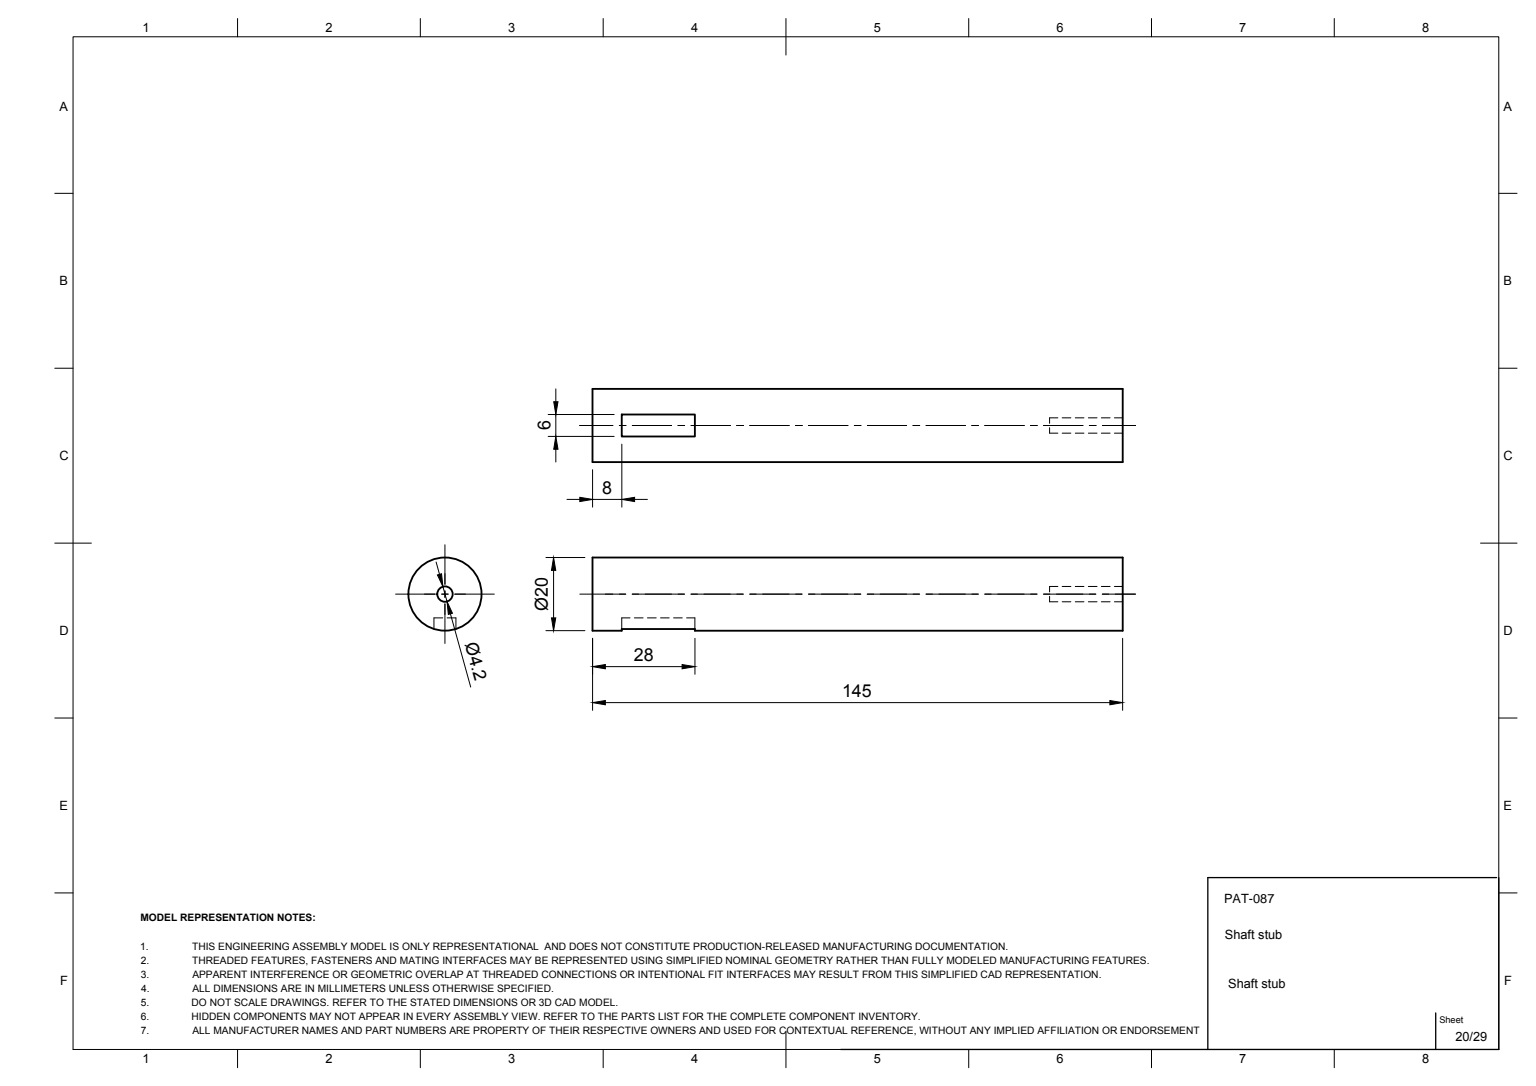
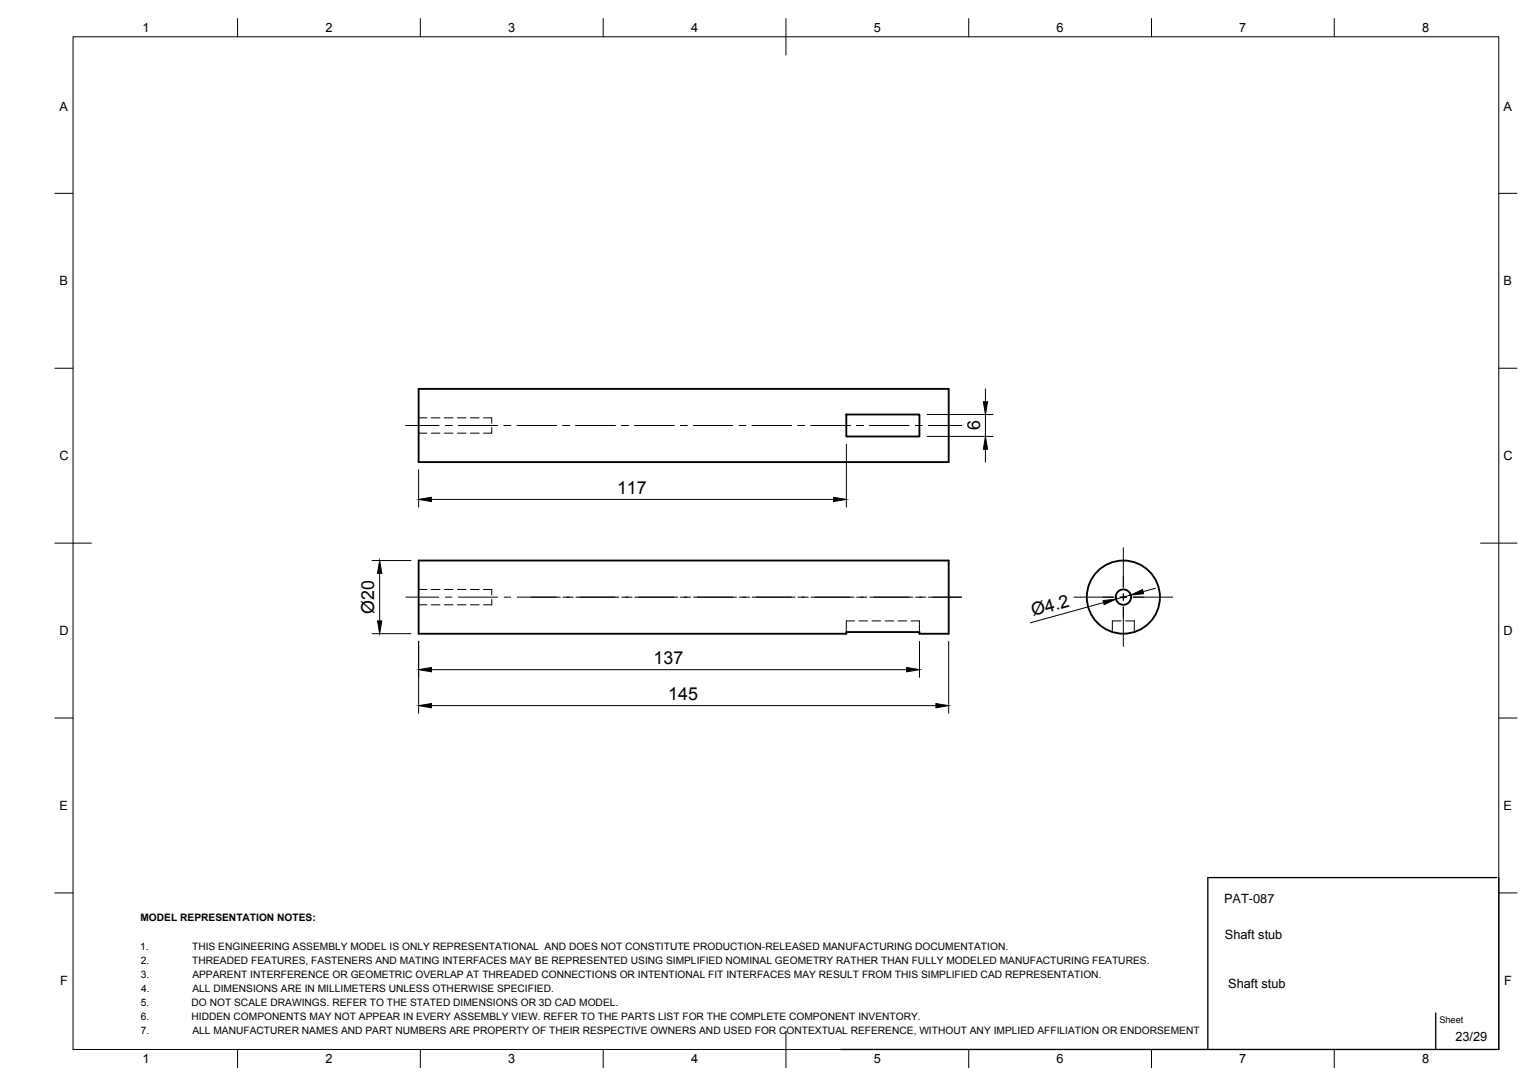
ISO-10303-21;
HEADER;
/* Generated by software containing ST-Developer
 * from STEP Tools, Inc. (www.steptools.com) 
 */

FILE_DESCRIPTION(
/* description */ ('Rigid flange shaft coupling assembly'),
/* implementation_level */ '2;1');

FILE_NAME(
/* name */ 'Shaft stub.step',
/* time_stamp */ '2026-10-27T10:47:16-07:00',
/* author */ (''),
/* organization */ (''),
/* preprocessor_version */ 'ST-DEVELOPER v20.2',
/* originating_system */ 'Autodesk Translation Framework v15.17.0.0',
/* authorisation */ '');

FILE_SCHEMA (('AUTOMOTIVE_DESIGN { 1 0 10303 214 3 1 1 }'));
ENDSEC;

DATA;
#10=MECHANICAL_DESIGN_GEOMETRIC_PRESENTATION_REPRESENTATION('',(#412),#9141);
#355=SHAPE_REPRESENTATION_RELATIONSHIP('SRR','None',#9291,#383);
#383=ADVANCED_BREP_SHAPE_REPRESENTATION('',(#440),#9126);
#412=STYLED_ITEM('',(#9500),#440);
#440=MANIFOLD_SOLID_BREP('Body1',#4767);
#517=FACE_BOUND('',#1207,.T.);
#518=FACE_BOUND('',#1210,.T.);
#645=PLANE('',#5312);
#646=PLANE('',#5313);
#647=PLANE('',#5314);
#648=PLANE('',#5316);
#649=PLANE('',#5317);
#650=PLANE('',#5318);
#651=PLANE('',#5323);
#652=PLANE('',#5324);
#863=FACE_OUTER_BOUND('',#1199,.T.);
#864=FACE_OUTER_BOUND('',#1200,.T.);
#865=FACE_OUTER_BOUND('',#1201,.T.);
#866=FACE_OUTER_BOUND('',#1202,.T.);
#867=FACE_OUTER_BOUND('',#1203,.T.);
#868=FACE_OUTER_BOUND('',#1204,.T.);
#869=FACE_OUTER_BOUND('',#1205,.T.);
#870=FACE_OUTER_BOUND('',#1206,.T.);
#871=FACE_OUTER_BOUND('',#1208,.T.);
#872=FACE_OUTER_BOUND('',#1209,.T.);
#1199=EDGE_LOOP('',(#3767,#3768,#3769,#3770));
#1200=EDGE_LOOP('',(#3771));
#1201=EDGE_LOOP('',(#3772,#3773,#3774,#3775));
#1202=EDGE_LOOP('',(#3776,#3777,#3778,#3779));
#1203=EDGE_LOOP('',(#3780,#3781,#3782,#3783));
#1204=EDGE_LOOP('',(#3784,#3785,#3786,#3787));
#1205=EDGE_LOOP('',(#3788,#3789,#3790,#3791));
#1206=EDGE_LOOP('',(#3792,#3793,#3794,#3795));
#1207=EDGE_LOOP('',(#3796,#3797,#3798,#3799));
#1208=EDGE_LOOP('',(#3800));
#1209=EDGE_LOOP('',(#3801));
#1210=EDGE_LOOP('',(#3802));
#1566=LINE('',#8079,#1911);
#1567=LINE('',#8085,#1912);
#1568=LINE('',#8087,#1913);
#1569=LINE('',#8089,#1914);
#1570=LINE('',#8090,#1915);
#1571=LINE('',#8095,#1916);
#1572=LINE('',#8096,#1917);
#1573=LINE('',#8099,#1918);
#1574=LINE('',#8101,#1919);
#1575=LINE('',#8102,#1920);
#1576=LINE('',#8104,#1921);
#1577=LINE('',#8111,#1922);
#1911=VECTOR('',#6239,0.21);
#1912=VECTOR('',#6246,1.);
#1913=VECTOR('',#6247,1.);
#1914=VECTOR('',#6248,1.);
#1915=VECTOR('',#6249,1.);
#1916=VECTOR('',#6254,1.);
#1917=VECTOR('',#6255,1.);
#1918=VECTOR('',#6258,1.);
#1919=VECTOR('',#6259,1.);
#1920=VECTOR('',#6260,1.);
#1921=VECTOR('',#6263,1.);
#1922=VECTOR('',#6272,1.);
#2172=CIRCLE('',#5310,0.21);
#2173=CIRCLE('',#5311,0.21);
#2174=CIRCLE('',#5315,1.);
#2175=CIRCLE('',#5319,1.);
#2176=CIRCLE('',#5321,1.);
#2177=CIRCLE('',#5322,1.);
#2457=VERTEX_POINT('',#8076);
#2458=VERTEX_POINT('',#8078);
#2459=VERTEX_POINT('',#8083);
#2460=VERTEX_POINT('',#8084);
#2461=VERTEX_POINT('',#8086);
#2462=VERTEX_POINT('',#8088);
#2463=VERTEX_POINT('',#8092);
#2464=VERTEX_POINT('',#8094);
#2465=VERTEX_POINT('',#8098);
#2466=VERTEX_POINT('',#8100);
#2467=VERTEX_POINT('',#8108);
#2468=VERTEX_POINT('',#8110);
#2927=EDGE_CURVE('',#2457,#2457,#2172,.T.);
#2928=EDGE_CURVE('',#2457,#2458,#1566,.T.);
#2929=EDGE_CURVE('',#2458,#2458,#2173,.T.);
#2930=EDGE_CURVE('',#2459,#2460,#1567,.T.);
#2931=EDGE_CURVE('',#2459,#2461,#1568,.T.);
#2932=EDGE_CURVE('',#2462,#2461,#1569,.T.);
#2933=EDGE_CURVE('',#2462,#2460,#1570,.T.);
#2934=EDGE_CURVE('',#2460,#2463,#2174,.T.);
#2935=EDGE_CURVE('',#2464,#2462,#1571,.T.);
#2936=EDGE_CURVE('',#2463,#2464,#1572,.T.);
#2937=EDGE_CURVE('',#2463,#2465,#1573,.T.);
#2938=EDGE_CURVE('',#2464,#2466,#1574,.T.);
#2939=EDGE_CURVE('',#2466,#2465,#1575,.T.);
#2940=EDGE_CURVE('',#2461,#2466,#1576,.T.);
#2941=EDGE_CURVE('',#2465,#2459,#2175,.T.);
#2942=EDGE_CURVE('',#2467,#2467,#2176,.T.);
#2943=EDGE_CURVE('',#2467,#2468,#1577,.T.);
#2944=EDGE_CURVE('',#2468,#2468,#2177,.T.);
#3767=ORIENTED_EDGE('',*,*,#2927,.F.);
#3768=ORIENTED_EDGE('',*,*,#2928,.T.);
#3769=ORIENTED_EDGE('',*,*,#2929,.T.);
#3770=ORIENTED_EDGE('',*,*,#2928,.F.);
#3771=ORIENTED_EDGE('',*,*,#2929,.F.);
#3772=ORIENTED_EDGE('',*,*,#2930,.F.);
#3773=ORIENTED_EDGE('',*,*,#2931,.T.);
#3774=ORIENTED_EDGE('',*,*,#2932,.F.);
#3775=ORIENTED_EDGE('',*,*,#2933,.T.);
#3776=ORIENTED_EDGE('',*,*,#2934,.F.);
#3777=ORIENTED_EDGE('',*,*,#2933,.F.);
#3778=ORIENTED_EDGE('',*,*,#2935,.F.);
#3779=ORIENTED_EDGE('',*,*,#2936,.F.);
#3780=ORIENTED_EDGE('',*,*,#2937,.F.);
#3781=ORIENTED_EDGE('',*,*,#2936,.T.);
#3782=ORIENTED_EDGE('',*,*,#2938,.T.);
#3783=ORIENTED_EDGE('',*,*,#2939,.T.);
#3784=ORIENTED_EDGE('',*,*,#2935,.T.);
#3785=ORIENTED_EDGE('',*,*,#2932,.T.);
#3786=ORIENTED_EDGE('',*,*,#2940,.T.);
#3787=ORIENTED_EDGE('',*,*,#2938,.F.);
#3788=ORIENTED_EDGE('',*,*,#2941,.F.);
#3789=ORIENTED_EDGE('',*,*,#2939,.F.);
#3790=ORIENTED_EDGE('',*,*,#2940,.F.);
#3791=ORIENTED_EDGE('',*,*,#2931,.F.);
#3792=ORIENTED_EDGE('',*,*,#2942,.F.);
#3793=ORIENTED_EDGE('',*,*,#2943,.T.);
#3794=ORIENTED_EDGE('',*,*,#2944,.T.);
#3795=ORIENTED_EDGE('',*,*,#2943,.F.);
#3796=ORIENTED_EDGE('',*,*,#2937,.T.);
#3797=ORIENTED_EDGE('',*,*,#2941,.T.);
#3798=ORIENTED_EDGE('',*,*,#2930,.T.);
#3799=ORIENTED_EDGE('',*,*,#2934,.T.);
#3800=ORIENTED_EDGE('',*,*,#2942,.T.);
#3801=ORIENTED_EDGE('',*,*,#2944,.F.);
#3802=ORIENTED_EDGE('',*,*,#2927,.T.);
#4438=CYLINDRICAL_SURFACE('',#5309,0.21);
#4439=CYLINDRICAL_SURFACE('',#5320,1.);
#4599=ADVANCED_FACE('',(#863),#4438,.F.);
#4600=ADVANCED_FACE('',(#864),#645,.F.);
#4601=ADVANCED_FACE('',(#865),#646,.F.);
#4602=ADVANCED_FACE('',(#866),#647,.T.);
#4603=ADVANCED_FACE('',(#867),#648,.F.);
#4604=ADVANCED_FACE('',(#868),#649,.F.);
#4605=ADVANCED_FACE('',(#869),#650,.F.);
#4606=ADVANCED_FACE('',(#870,#517),#4439,.T.);
#4607=ADVANCED_FACE('',(#871),#651,.T.);
#4608=ADVANCED_FACE('',(#872,#518),#652,.F.);
#4767=CLOSED_SHELL('',(#4599,#4600,#4601,#4602,#4603,#4604,#4605,#4606,
#4607,#4608));
#5308=AXIS2_PLACEMENT_3D('',#8074,#6233,#6234);
#5309=AXIS2_PLACEMENT_3D('',#8075,#6235,#6236);
#5310=AXIS2_PLACEMENT_3D('',#8077,#6237,#6238);
#5311=AXIS2_PLACEMENT_3D('',#8080,#6240,#6241);
#5312=AXIS2_PLACEMENT_3D('',#8081,#6242,#6243);
#5313=AXIS2_PLACEMENT_3D('',#8082,#6244,#6245);
#5314=AXIS2_PLACEMENT_3D('',#8091,#6250,#6251);
#5315=AXIS2_PLACEMENT_3D('',#8093,#6252,#6253);
#5316=AXIS2_PLACEMENT_3D('',#8097,#6256,#6257);
#5317=AXIS2_PLACEMENT_3D('',#8103,#6261,#6262);
#5318=AXIS2_PLACEMENT_3D('',#8105,#6264,#6265);
#5319=AXIS2_PLACEMENT_3D('',#8106,#6266,#6267);
#5320=AXIS2_PLACEMENT_3D('',#8107,#6268,#6269);
#5321=AXIS2_PLACEMENT_3D('',#8109,#6270,#6271);
#5322=AXIS2_PLACEMENT_3D('',#8112,#6273,#6274);
#5323=AXIS2_PLACEMENT_3D('',#8113,#6275,#6276);
#5324=AXIS2_PLACEMENT_3D('',#8114,#6277,#6278);
#6233=DIRECTION('axis',(0.,0.,1.));
#6234=DIRECTION('refdir',(1.,0.,0.));
#6235=DIRECTION('center_axis',(0.,1.,0.));
#6236=DIRECTION('ref_axis',(1.,0.,0.));
#6237=DIRECTION('center_axis',(0.,1.,0.));
#6238=DIRECTION('ref_axis',(1.,0.,0.));
#6239=DIRECTION('',(0.,1.,0.));
#6240=DIRECTION('center_axis',(0.,1.,0.));
#6241=DIRECTION('ref_axis',(1.,0.,0.));
#6242=DIRECTION('center_axis',(0.,1.,0.));
#6243=DIRECTION('ref_axis',(1.,0.,0.));
#6244=DIRECTION('center_axis',(-1.,0.,0.));
#6245=DIRECTION('ref_axis',(0.,0.,1.));
#6246=DIRECTION('',(0.,-1.,0.));
#6247=DIRECTION('',(0.,0.,1.));
#6248=DIRECTION('',(0.,1.,0.));
#6249=DIRECTION('',(0.,0.,-1.));
#6250=DIRECTION('center_axis',(0.,1.,0.));
#6251=DIRECTION('ref_axis',(1.,0.,0.));
#6252=DIRECTION('center_axis',(0.,-1.,0.));
#6253=DIRECTION('ref_axis',(1.,0.,0.));
#6254=DIRECTION('',(-1.,0.,0.));
#6255=DIRECTION('',(0.,0.,1.));
#6256=DIRECTION('center_axis',(1.,0.,0.));
#6257=DIRECTION('ref_axis',(0.,0.,-1.));
#6258=DIRECTION('',(0.,1.,0.));
#6259=DIRECTION('',(0.,1.,0.));
#6260=DIRECTION('',(0.,0.,-1.));
#6261=DIRECTION('center_axis',(0.,0.,1.));
#6262=DIRECTION('ref_axis',(1.,0.,0.));
#6263=DIRECTION('',(1.,0.,0.));
#6264=DIRECTION('center_axis',(0.,1.,0.));
#6265=DIRECTION('ref_axis',(0.,0.,1.));
#6266=DIRECTION('center_axis',(0.,1.,0.));
#6267=DIRECTION('ref_axis',(1.,0.,0.));
#6268=DIRECTION('center_axis',(0.,1.,0.));
#6269=DIRECTION('ref_axis',(1.,0.,0.));
#6270=DIRECTION('center_axis',(0.,1.,0.));
#6271=DIRECTION('ref_axis',(1.,0.,0.));
#6272=DIRECTION('',(0.,-1.,0.));
#6273=DIRECTION('center_axis',(0.,1.,0.));
#6274=DIRECTION('ref_axis',(1.,0.,0.));
#6275=DIRECTION('center_axis',(0.,1.,0.));
#6276=DIRECTION('ref_axis',(1.,0.,0.));
#6277=DIRECTION('center_axis',(0.,1.,0.));
#6278=DIRECTION('ref_axis',(1.,0.,0.));
#8074=CARTESIAN_POINT('',(0.,0.,0.));
#8075=CARTESIAN_POINT('Origin',(0.,-4.6,6.53));
#8076=CARTESIAN_POINT('',(-0.21,-4.5,6.53));
#8077=CARTESIAN_POINT('Origin',(0.,-4.5,6.53));
#8078=CARTESIAN_POINT('',(-0.21,-2.5,6.53));
#8079=CARTESIAN_POINT('',(-0.21,-4.6,6.53));
#8080=CARTESIAN_POINT('Origin',(0.,-2.5,6.53));
#8081=CARTESIAN_POINT('Origin',(0.,-2.5,6.53));
#8082=CARTESIAN_POINT('Origin',(-0.3,7.2,5.43));
#8083=CARTESIAN_POINT('',(-0.3,9.2,5.57606079858305));
#8084=CARTESIAN_POINT('',(-0.3,7.2,5.57606079858305));
#8085=CARTESIAN_POINT('',(-0.3,-4.5,5.57606079858305));
#8086=CARTESIAN_POINT('',(-0.3,9.2,5.88));
#8087=CARTESIAN_POINT('',(-0.3,9.2,5.88));
#8088=CARTESIAN_POINT('',(-0.3,7.2,5.88));
#8089=CARTESIAN_POINT('',(-0.3,7.2,5.88));
#8090=CARTESIAN_POINT('',(-0.3,7.2,5.88));
#8091=CARTESIAN_POINT('Origin',(0.,7.2,5.655));
#8092=CARTESIAN_POINT('',(0.3,7.2,5.57606079858305));
#8093=CARTESIAN_POINT('Origin',(0.,7.2,6.53));
#8094=CARTESIAN_POINT('',(0.3,7.2,5.88));
#8095=CARTESIAN_POINT('',(0.3,7.2,5.88));
#8096=CARTESIAN_POINT('',(0.3,7.2,5.43));
#8097=CARTESIAN_POINT('Origin',(0.3,7.2,5.88));
#8098=CARTESIAN_POINT('',(0.3,9.2,5.57606079858305));
#8099=CARTESIAN_POINT('',(0.3,-4.5,5.57606079858305));
#8100=CARTESIAN_POINT('',(0.3,9.2,5.88));
#8101=CARTESIAN_POINT('',(0.3,7.2,5.88));
#8102=CARTESIAN_POINT('',(0.3,9.2,5.43));
#8103=CARTESIAN_POINT('Origin',(-0.3,7.2,5.88));
#8104=CARTESIAN_POINT('',(0.3,9.2,5.88));
#8105=CARTESIAN_POINT('Origin',(0.,9.2,5.655));
#8106=CARTESIAN_POINT('Origin',(0.,9.2,6.53));
#8107=CARTESIAN_POINT('Origin',(0.,-4.5,6.53));
#8108=CARTESIAN_POINT('',(-1.,10.,6.53));
#8109=CARTESIAN_POINT('Origin',(0.,10.,6.53));
#8110=CARTESIAN_POINT('',(-1.,-4.5,6.53));
#8111=CARTESIAN_POINT('',(-1.,-4.5,6.53));
#8112=CARTESIAN_POINT('Origin',(0.,-4.5,6.53));
#8113=CARTESIAN_POINT('Origin',(0.,10.,6.53));
#8114=CARTESIAN_POINT('Origin',(0.,-4.5,6.53));
#9093=UNCERTAINTY_MEASURE_WITH_UNIT(LENGTH_MEASURE(0.001),#9142,
'DISTANCE_ACCURACY_VALUE',
'Maximum model space distance between geometric entities at asserted c
onnectivities');
#9108=UNCERTAINTY_MEASURE_WITH_UNIT(LENGTH_MEASURE(0.001),#9142,
'DISTANCE_ACCURACY_VALUE',
'Maximum model space distance between geometric entities at asserted c
onnectivities');
#9126=(
GEOMETRIC_REPRESENTATION_CONTEXT(3)
GLOBAL_UNCERTAINTY_ASSIGNED_CONTEXT((#9093))
GLOBAL_UNIT_ASSIGNED_CONTEXT((#9142,#9144,#9145))
REPRESENTATION_CONTEXT('','3D')
);
#9141=(
GEOMETRIC_REPRESENTATION_CONTEXT(3)
GLOBAL_UNCERTAINTY_ASSIGNED_CONTEXT((#9108))
GLOBAL_UNIT_ASSIGNED_CONTEXT((#9142,#9144,#9145))
REPRESENTATION_CONTEXT('','3D')
);
#9142=(
LENGTH_UNIT()
NAMED_UNIT(*)
SI_UNIT(.CENTI.,.METRE.)
);
#9144=(
NAMED_UNIT(*)
PLANE_ANGLE_UNIT()
SI_UNIT($,.RADIAN.)
);
#9145=(
NAMED_UNIT(*)
SI_UNIT($,.STERADIAN.)
SOLID_ANGLE_UNIT()
);
#9163=SHAPE_DEFINITION_REPRESENTATION(#9197,#9291);
#9197=PRODUCT_DEFINITION_SHAPE('',$,#9324);
#9291=SHAPE_REPRESENTATION('',(#5308),#9126);
#9306=PRODUCT_DEFINITION_CONTEXT('part definition',#9404,'design');
#9324=PRODUCT_DEFINITION('Shaft stub','Shaft stub',#9356,#9306);
#9356=PRODUCT_DEFINITION_FORMATION('',$,#9423);
#9404=APPLICATION_CONTEXT(
'Core Data for Automotive Mechanical Design Process');
#9405=PRODUCT_CONTEXT('part definition',#9404,'mechanical');
#9423=PRODUCT('Shaft stub','Shaft stub','Shaft stub',(#9405));
#9494=COLOUR_RGB('Grey',0.48,0.52,0.57);
#9495=FILL_AREA_STYLE_COLOUR('',#9494);
#9496=FILL_AREA_STYLE('',(#9495));
#9497=SURFACE_STYLE_FILL_AREA(#9496);
#9498=SURFACE_SIDE_STYLE('',(#9497));
#9499=SURFACE_STYLE_USAGE(.BOTH.,#9498);
#9500=PRESENTATION_STYLE_ASSIGNMENT((#9499));
ENDSEC;
END-ISO-10303-21;
